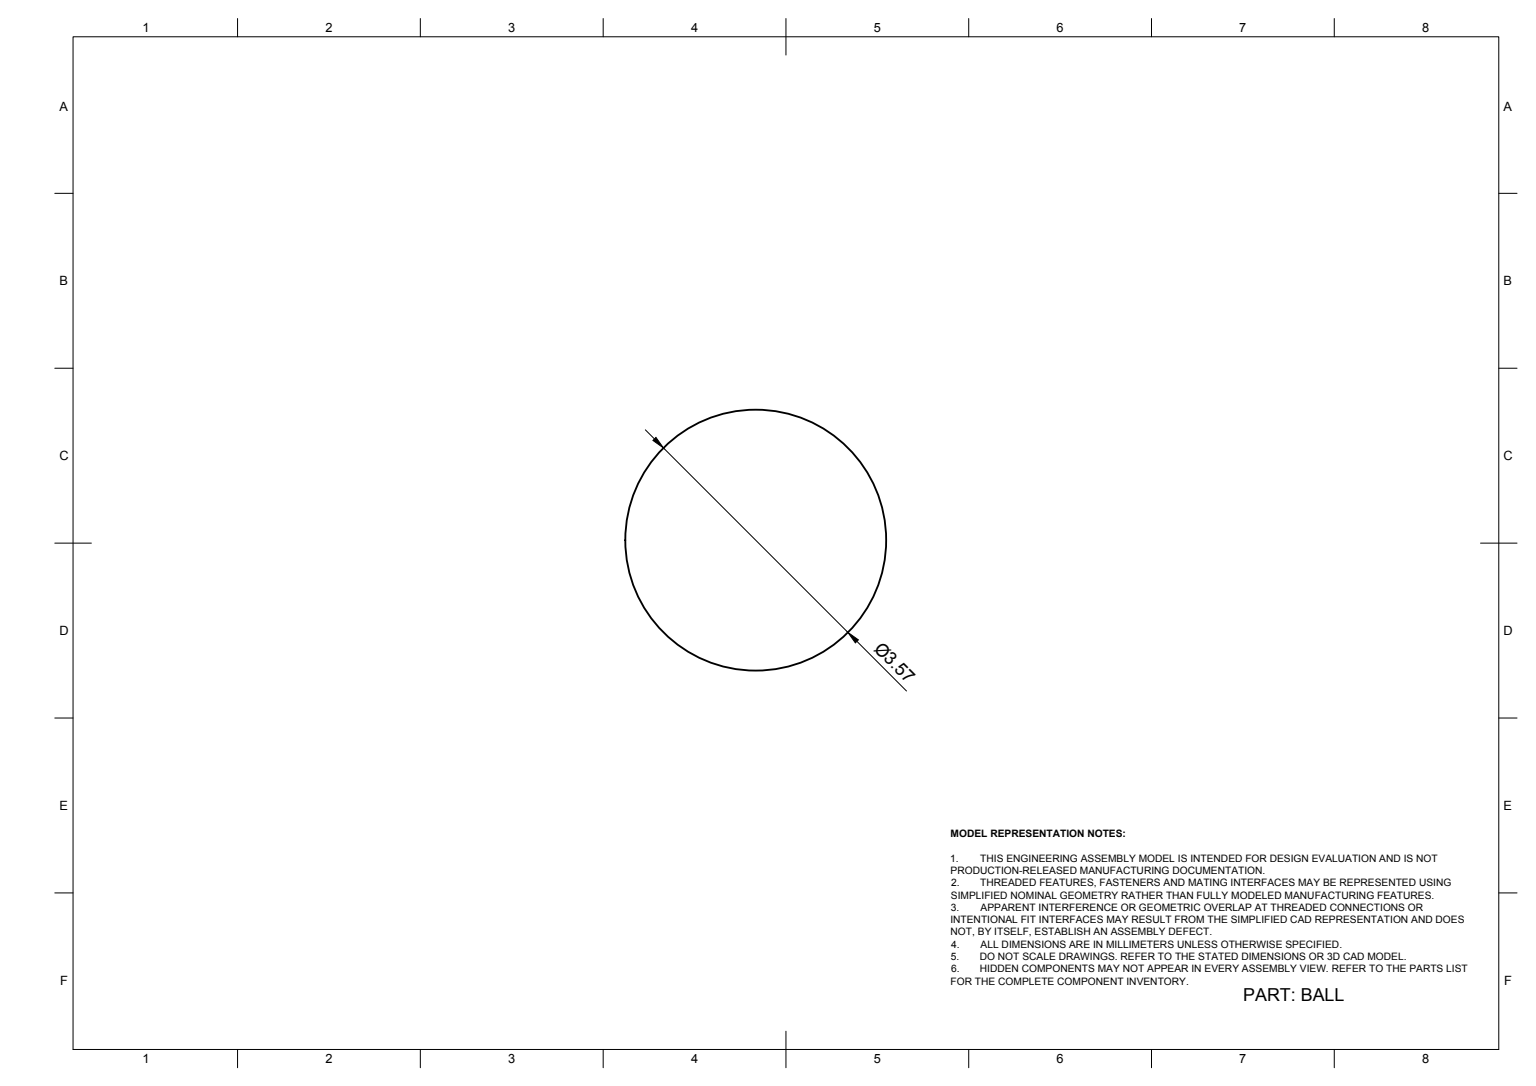
ISO-10303-21;
HEADER;
/* Generated by software containing ST-Developer
 * from STEP Tools, Inc. (www.steptools.com) 
 */

FILE_DESCRIPTION(
/* description */ (''),
/* implementation_level */ '2;1');

FILE_NAME(
/* name */ 'Ball.step',
/* time_stamp */ '2026-10-05T00:51:14-07:00',
/* author */ (''),
/* organization */ (''),
/* preprocessor_version */ 'ST-DEVELOPER v20.2',
/* originating_system */ 'Autodesk Translation Framework v15.15.0.0',
/* authorisation */ '');

FILE_SCHEMA (('AUTOMOTIVE_DESIGN { 1 0 10303 214 3 1 1 }'));
ENDSEC;

DATA;
#10=MECHANICAL_DESIGN_GEOMETRIC_PRESENTATION_REPRESENTATION('',(#387),#4613);
#371=SHAPE_REPRESENTATION_RELATIONSHIP('SRR','None',#4645,#379);
#379=ADVANCED_BREP_SHAPE_REPRESENTATION('',(#395),#4605);
#387=STYLED_ITEM('',(#4694),#395);
#395=MANIFOLD_SOLID_BREP('Body1',#1594);
#403=FACE_OUTER_BOUND('',#509,.T.);
#509=EDGE_LOOP('',(#1071,#1072));
#639=CIRCLE('',#1694,1.78305659323844);
#731=VERTEX_POINT('',#2410);
#732=VERTEX_POINT('',#2411);
#863=EDGE_CURVE('',#731,#732,#639,.T.);
#1071=ORIENTED_EDGE('',*,*,#863,.T.);
#1072=ORIENTED_EDGE('',*,*,#863,.F.);
#1487=SPHERICAL_SURFACE('',#1693,1.78305659323844);
#1488=ADVANCED_FACE('',(#403),#1487,.T.);
#1594=CLOSED_SHELL('',(#1488));
#1692=AXIS2_PLACEMENT_3D('',#2408,#1904,#1905);
#1693=AXIS2_PLACEMENT_3D('',#2409,#1906,#1907);
#1694=AXIS2_PLACEMENT_3D('',#2412,#1908,#1909);
#1904=DIRECTION('axis',(0.,0.,1.));
#1905=DIRECTION('refdir',(1.,0.,0.));
#1906=DIRECTION('center_axis',(1.,-1.22464679914735E-16,0.));
#1907=DIRECTION('ref_axis',(0.,-1.,0.));
#1908=DIRECTION('center_axis',(-7.49879891330929E-33,-1.22464679914735E-16,
1.));
#1909=DIRECTION('ref_axis',(0.,1.,1.22464679914735E-16));
#2408=CARTESIAN_POINT('',(0.,0.,0.));
#2409=CARTESIAN_POINT('Origin',(-28.33623852117,0.,0.));
#2410=CARTESIAN_POINT('',(-26.5531819279316,1.09180727480402E-16,2.67415656874908E-32));
#2411=CARTESIAN_POINT('',(-30.1192951144084,1.09180727480402E-16,-6.84227765783602E-48));
#2412=CARTESIAN_POINT('Origin',(-28.33623852117,0.,0.));
#4595=UNCERTAINTY_MEASURE_WITH_UNIT(LENGTH_MEASURE(0.01),#4614,
'DISTANCE_ACCURACY_VALUE',
'Maximum model space distance between geometric entities at asserted c
onnectivities');
#4603=UNCERTAINTY_MEASURE_WITH_UNIT(LENGTH_MEASURE(0.01),#4614,
'DISTANCE_ACCURACY_VALUE',
'Maximum model space distance between geometric entities at asserted c
onnectivities');
#4605=(
GEOMETRIC_REPRESENTATION_CONTEXT(3)
GLOBAL_UNCERTAINTY_ASSIGNED_CONTEXT((#4595))
GLOBAL_UNIT_ASSIGNED_CONTEXT((#4614,#4616,#4617))
REPRESENTATION_CONTEXT('','3D')
);
#4613=(
GEOMETRIC_REPRESENTATION_CONTEXT(3)
GLOBAL_UNCERTAINTY_ASSIGNED_CONTEXT((#4603))
GLOBAL_UNIT_ASSIGNED_CONTEXT((#4614,#4616,#4617))
REPRESENTATION_CONTEXT('','3D')
);
#4614=(
LENGTH_UNIT()
NAMED_UNIT(*)
SI_UNIT(.MILLI.,.METRE.)
);
#4616=(
NAMED_UNIT(*)
PLANE_ANGLE_UNIT()
SI_UNIT($,.RADIAN.)
);
#4617=(
NAMED_UNIT(*)
SI_UNIT($,.STERADIAN.)
SOLID_ANGLE_UNIT()
);
#4619=SHAPE_DEFINITION_REPRESENTATION(#4628,#4645);
#4628=PRODUCT_DEFINITION_SHAPE('',$,#4655);
#4645=SHAPE_REPRESENTATION('',(#1692),#4605);
#4653=PRODUCT_DEFINITION_CONTEXT('part definition',#4682,'design');
#4655=PRODUCT_DEFINITION('Ball','Ball',#4664,#4653);
#4664=PRODUCT_DEFINITION_FORMATION('',$,#4685);
#4682=APPLICATION_CONTEXT(
'Core Data for Automotive Mechanical Design Process');
#4683=PRODUCT_CONTEXT('part definition',#4682,'mechanical');
#4685=PRODUCT('Ball','Ball',$,(#4683));
#4694=PRESENTATION_STYLE_ASSIGNMENT((#4699));
#4699=SURFACE_STYLE_USAGE(.BOTH.,#4704);
#4704=SURFACE_SIDE_STYLE('',(#4709));
#4709=SURFACE_STYLE_FILL_AREA(#4714);
#4714=FILL_AREA_STYLE('Opaque(170,85,127)',(#4719));
#4719=FILL_AREA_STYLE_COLOUR('Opaque(170,85,127)',#4724);
#4724=COLOUR_RGB('Opaque(170,85,127)', 0.09019608, 0.27058824, 0.51372549);
ENDSEC;
END-ISO-10303-21;
